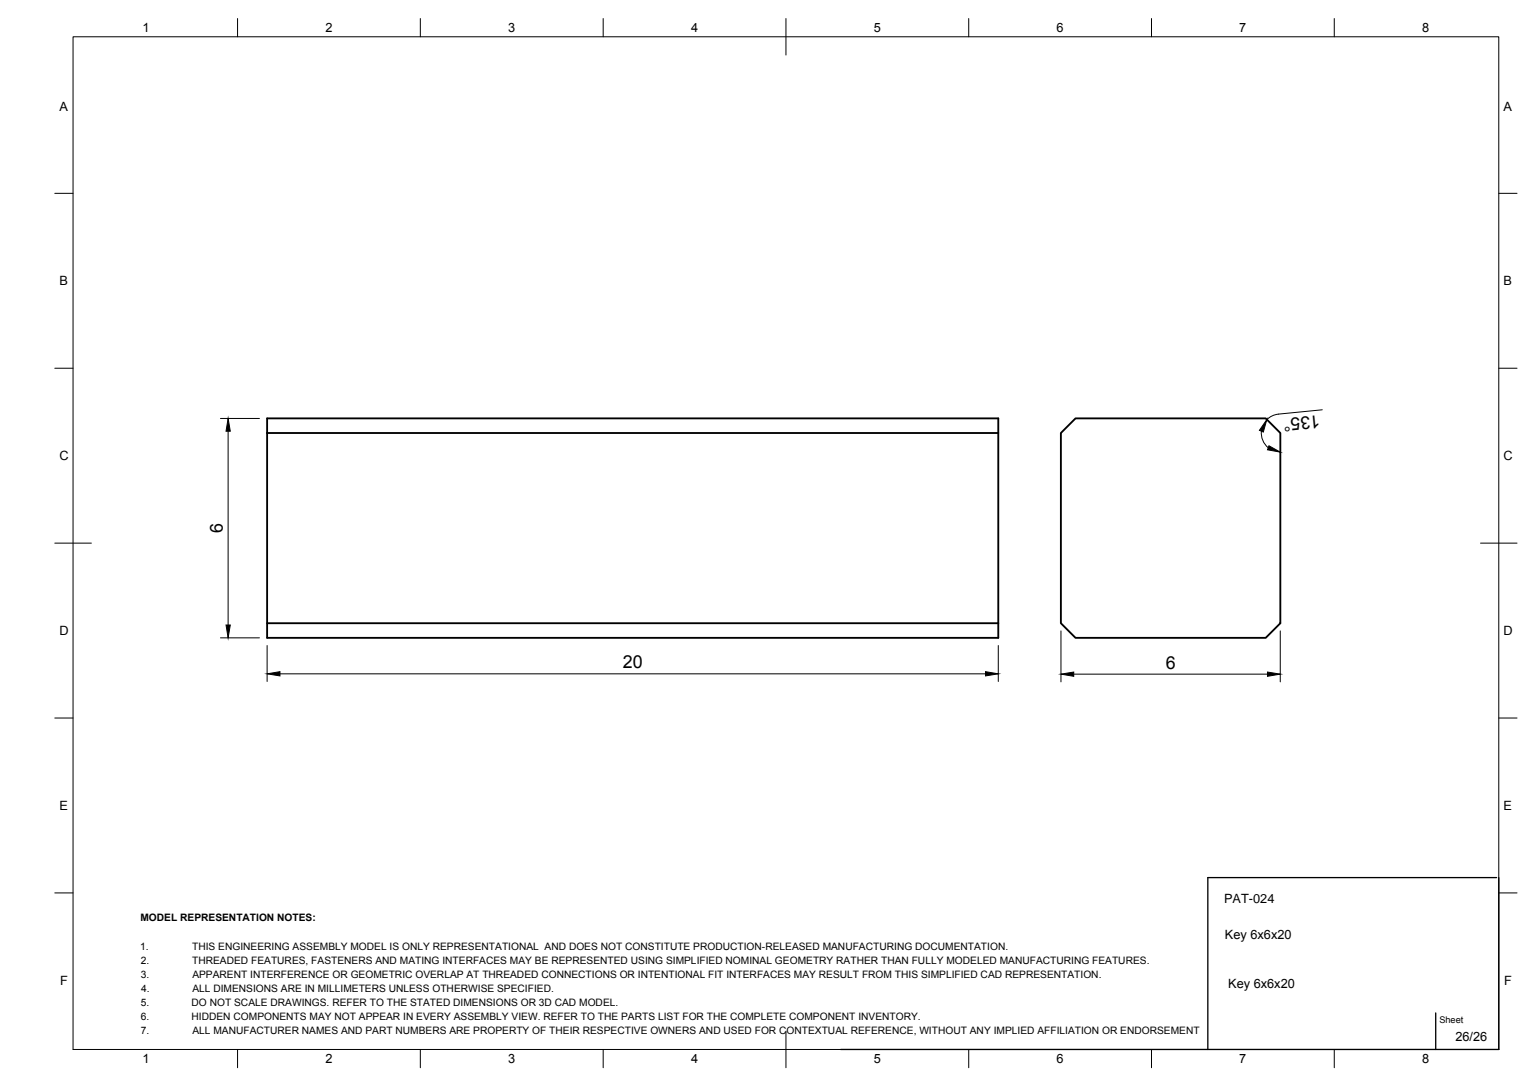
ISO-10303-21;
HEADER;
/* Generated by software containing ST-Developer
 * from STEP Tools, Inc. (www.steptools.com) 
 */

FILE_DESCRIPTION(
/* description */ ('Compact handwheel screw vise'),
/* implementation_level */ '2;1');

FILE_NAME(
/* name */ 'Key 6x6x20.step',
/* time_stamp */ '2026-10-29T16:08:22-07:00',
/* author */ (''),
/* organization */ (''),
/* preprocessor_version */ 'ST-DEVELOPER v20.2',
/* originating_system */ 'Autodesk Translation Framework v15.17.0.0',
/* authorisation */ '');

FILE_SCHEMA (('AUTOMOTIVE_DESIGN { 1 0 10303 214 3 1 1 }'));
ENDSEC;

DATA;
#10=MECHANICAL_DESIGN_GEOMETRIC_PRESENTATION_REPRESENTATION('',(#676),#25074);
#612=SHAPE_REPRESENTATION_RELATIONSHIP('SRR','None',#25223,#640);
#640=ADVANCED_BREP_SHAPE_REPRESENTATION('',(#709),#25070);
#676=STYLED_ITEM('',(#25439),#709);
#709=MANIFOLD_SOLID_BREP('Body1',#8087);
#980=PLANE('',#9109);
#981=PLANE('',#9110);
#982=PLANE('',#9111);
#983=PLANE('',#9112);
#984=PLANE('',#9113);
#985=PLANE('',#9114);
#986=PLANE('',#9115);
#987=PLANE('',#9116);
#988=PLANE('',#9117);
#989=PLANE('',#9118);
#1439=FACE_OUTER_BOUND('',#2015,.T.);
#1440=FACE_OUTER_BOUND('',#2016,.T.);
#1441=FACE_OUTER_BOUND('',#2017,.T.);
#1442=FACE_OUTER_BOUND('',#2018,.T.);
#1443=FACE_OUTER_BOUND('',#2019,.T.);
#1444=FACE_OUTER_BOUND('',#2020,.T.);
#1445=FACE_OUTER_BOUND('',#2021,.T.);
#1446=FACE_OUTER_BOUND('',#2022,.T.);
#1447=FACE_OUTER_BOUND('',#2023,.T.);
#1448=FACE_OUTER_BOUND('',#2024,.T.);
#2015=EDGE_LOOP('',(#7171,#7172,#7173,#7174,#7175,#7176,#7177,#7178));
#2016=EDGE_LOOP('',(#7179,#7180,#7181,#7182));
#2017=EDGE_LOOP('',(#7183,#7184,#7185,#7186));
#2018=EDGE_LOOP('',(#7187,#7188,#7189,#7190));
#2019=EDGE_LOOP('',(#7191,#7192,#7193,#7194));
#2020=EDGE_LOOP('',(#7195,#7196,#7197,#7198,#7199,#7200,#7201,#7202));
#2021=EDGE_LOOP('',(#7203,#7204,#7205,#7206));
#2022=EDGE_LOOP('',(#7207,#7208,#7209,#7210));
#2023=EDGE_LOOP('',(#7211,#7212,#7213,#7214));
#2024=EDGE_LOOP('',(#7215,#7216,#7217,#7218));
#2499=LINE('',#24788,#3007);
#2500=LINE('',#24790,#3008);
#2501=LINE('',#24792,#3009);
#2502=LINE('',#24794,#3010);
#2503=LINE('',#24796,#3011);
#2504=LINE('',#24798,#3012);
#2505=LINE('',#24800,#3013);
#2506=LINE('',#24801,#3014);
#2507=LINE('',#24804,#3015);
#2508=LINE('',#24806,#3016);
#2509=LINE('',#24807,#3017);
#2510=LINE('',#24810,#3018);
#2511=LINE('',#24811,#3019);
#2512=LINE('',#24814,#3020);
#2513=LINE('',#24815,#3021);
#2514=LINE('',#24818,#3022);
#2515=LINE('',#24819,#3023);
#2516=LINE('',#24823,#3024);
#2517=LINE('',#24824,#3025);
#2518=LINE('',#24826,#3026);
#2519=LINE('',#24827,#3027);
#2520=LINE('',#24829,#3028);
#2521=LINE('',#24831,#3029);
#2522=LINE('',#24833,#3030);
#3007=VECTOR('',#11059,1.);
#3008=VECTOR('',#11060,1.);
#3009=VECTOR('',#11061,1.);
#3010=VECTOR('',#11062,1.);
#3011=VECTOR('',#11063,1.);
#3012=VECTOR('',#11064,1.);
#3013=VECTOR('',#11065,1.);
#3014=VECTOR('',#11066,1.);
#3015=VECTOR('',#11069,1.);
#3016=VECTOR('',#11070,1.);
#3017=VECTOR('',#11071,1.);
#3018=VECTOR('',#11074,1.);
#3019=VECTOR('',#11075,1.);
#3020=VECTOR('',#11078,1.);
#3021=VECTOR('',#11079,1.);
#3022=VECTOR('',#11082,1.);
#3023=VECTOR('',#11083,1.);
#3024=VECTOR('',#11086,1.);
#3025=VECTOR('',#11087,1.);
#3026=VECTOR('',#11088,1.);
#3027=VECTOR('',#11089,1.);
#3028=VECTOR('',#11092,1.);
#3029=VECTOR('',#11095,1.);
#3030=VECTOR('',#11098,1.);
#4010=VERTEX_POINT('',#24786);
#4011=VERTEX_POINT('',#24787);
#4012=VERTEX_POINT('',#24789);
#4013=VERTEX_POINT('',#24791);
#4014=VERTEX_POINT('',#24793);
#4015=VERTEX_POINT('',#24795);
#4016=VERTEX_POINT('',#24797);
#4017=VERTEX_POINT('',#24799);
#4018=VERTEX_POINT('',#24803);
#4019=VERTEX_POINT('',#24805);
#4020=VERTEX_POINT('',#24809);
#4021=VERTEX_POINT('',#24813);
#4022=VERTEX_POINT('',#24817);
#4023=VERTEX_POINT('',#24821);
#4024=VERTEX_POINT('',#24822);
#4025=VERTEX_POINT('',#24825);
#5072=EDGE_CURVE('',#4010,#4011,#2499,.T.);
#5073=EDGE_CURVE('',#4012,#4010,#2500,.T.);
#5074=EDGE_CURVE('',#4013,#4012,#2501,.T.);
#5075=EDGE_CURVE('',#4014,#4013,#2502,.T.);
#5076=EDGE_CURVE('',#4015,#4014,#2503,.T.);
#5077=EDGE_CURVE('',#4016,#4015,#2504,.T.);
#5078=EDGE_CURVE('',#4017,#4016,#2505,.T.);
#5079=EDGE_CURVE('',#4011,#4017,#2506,.T.);
#5080=EDGE_CURVE('',#4014,#4018,#2507,.T.);
#5081=EDGE_CURVE('',#4018,#4019,#2508,.T.);
#5082=EDGE_CURVE('',#4019,#4015,#2509,.T.);
#5083=EDGE_CURVE('',#4020,#4013,#2510,.T.);
#5084=EDGE_CURVE('',#4020,#4018,#2511,.T.);
#5085=EDGE_CURVE('',#4012,#4021,#2512,.T.);
#5086=EDGE_CURVE('',#4021,#4020,#2513,.T.);
#5087=EDGE_CURVE('',#4022,#4010,#2514,.T.);
#5088=EDGE_CURVE('',#4022,#4021,#2515,.T.);
#5089=EDGE_CURVE('',#4023,#4024,#2516,.T.);
#5090=EDGE_CURVE('',#4019,#4023,#2517,.T.);
#5091=EDGE_CURVE('',#4025,#4022,#2518,.T.);
#5092=EDGE_CURVE('',#4024,#4025,#2519,.T.);
#5093=EDGE_CURVE('',#4016,#4023,#2520,.T.);
#5094=EDGE_CURVE('',#4011,#4025,#2521,.T.);
#5095=EDGE_CURVE('',#4024,#4017,#2522,.T.);
#7171=ORIENTED_EDGE('',*,*,#5072,.F.);
#7172=ORIENTED_EDGE('',*,*,#5073,.F.);
#7173=ORIENTED_EDGE('',*,*,#5074,.F.);
#7174=ORIENTED_EDGE('',*,*,#5075,.F.);
#7175=ORIENTED_EDGE('',*,*,#5076,.F.);
#7176=ORIENTED_EDGE('',*,*,#5077,.F.);
#7177=ORIENTED_EDGE('',*,*,#5078,.F.);
#7178=ORIENTED_EDGE('',*,*,#5079,.F.);
#7179=ORIENTED_EDGE('',*,*,#5076,.T.);
#7180=ORIENTED_EDGE('',*,*,#5080,.T.);
#7181=ORIENTED_EDGE('',*,*,#5081,.T.);
#7182=ORIENTED_EDGE('',*,*,#5082,.T.);
#7183=ORIENTED_EDGE('',*,*,#5075,.T.);
#7184=ORIENTED_EDGE('',*,*,#5083,.F.);
#7185=ORIENTED_EDGE('',*,*,#5084,.T.);
#7186=ORIENTED_EDGE('',*,*,#5080,.F.);
#7187=ORIENTED_EDGE('',*,*,#5074,.T.);
#7188=ORIENTED_EDGE('',*,*,#5085,.T.);
#7189=ORIENTED_EDGE('',*,*,#5086,.T.);
#7190=ORIENTED_EDGE('',*,*,#5083,.T.);
#7191=ORIENTED_EDGE('',*,*,#5073,.T.);
#7192=ORIENTED_EDGE('',*,*,#5087,.F.);
#7193=ORIENTED_EDGE('',*,*,#5088,.T.);
#7194=ORIENTED_EDGE('',*,*,#5085,.F.);
#7195=ORIENTED_EDGE('',*,*,#5089,.F.);
#7196=ORIENTED_EDGE('',*,*,#5090,.F.);
#7197=ORIENTED_EDGE('',*,*,#5081,.F.);
#7198=ORIENTED_EDGE('',*,*,#5084,.F.);
#7199=ORIENTED_EDGE('',*,*,#5086,.F.);
#7200=ORIENTED_EDGE('',*,*,#5088,.F.);
#7201=ORIENTED_EDGE('',*,*,#5091,.F.);
#7202=ORIENTED_EDGE('',*,*,#5092,.F.);
#7203=ORIENTED_EDGE('',*,*,#5077,.T.);
#7204=ORIENTED_EDGE('',*,*,#5082,.F.);
#7205=ORIENTED_EDGE('',*,*,#5090,.T.);
#7206=ORIENTED_EDGE('',*,*,#5093,.F.);
#7207=ORIENTED_EDGE('',*,*,#5072,.T.);
#7208=ORIENTED_EDGE('',*,*,#5094,.T.);
#7209=ORIENTED_EDGE('',*,*,#5091,.T.);
#7210=ORIENTED_EDGE('',*,*,#5087,.T.);
#7211=ORIENTED_EDGE('',*,*,#5078,.T.);
#7212=ORIENTED_EDGE('',*,*,#5093,.T.);
#7213=ORIENTED_EDGE('',*,*,#5089,.T.);
#7214=ORIENTED_EDGE('',*,*,#5095,.T.);
#7215=ORIENTED_EDGE('',*,*,#5079,.T.);
#7216=ORIENTED_EDGE('',*,*,#5095,.F.);
#7217=ORIENTED_EDGE('',*,*,#5092,.T.);
#7218=ORIENTED_EDGE('',*,*,#5094,.F.);
#8009=ADVANCED_FACE('',(#1439),#980,.F.);
#8010=ADVANCED_FACE('',(#1440),#981,.T.);
#8011=ADVANCED_FACE('',(#1441),#982,.T.);
#8012=ADVANCED_FACE('',(#1442),#983,.T.);
#8013=ADVANCED_FACE('',(#1443),#984,.T.);
#8014=ADVANCED_FACE('',(#1444),#985,.T.);
#8015=ADVANCED_FACE('',(#1445),#986,.F.);
#8016=ADVANCED_FACE('',(#1446),#987,.T.);
#8017=ADVANCED_FACE('',(#1447),#988,.T.);
#8018=ADVANCED_FACE('',(#1448),#989,.T.);
#8087=CLOSED_SHELL('',(#8009,#8010,#8011,#8012,#8013,#8014,#8015,#8016,
#8017,#8018));
#9108=AXIS2_PLACEMENT_3D('',#24784,#11055,#11056);
#9109=AXIS2_PLACEMENT_3D('',#24785,#11057,#11058);
#9110=AXIS2_PLACEMENT_3D('',#24802,#11067,#11068);
#9111=AXIS2_PLACEMENT_3D('',#24808,#11072,#11073);
#9112=AXIS2_PLACEMENT_3D('',#24812,#11076,#11077);
#9113=AXIS2_PLACEMENT_3D('',#24816,#11080,#11081);
#9114=AXIS2_PLACEMENT_3D('',#24820,#11084,#11085);
#9115=AXIS2_PLACEMENT_3D('',#24828,#11090,#11091);
#9116=AXIS2_PLACEMENT_3D('',#24830,#11093,#11094);
#9117=AXIS2_PLACEMENT_3D('',#24832,#11096,#11097);
#9118=AXIS2_PLACEMENT_3D('',#24834,#11099,#11100);
#11055=DIRECTION('axis',(0.,0.,1.));
#11056=DIRECTION('refdir',(1.,0.,0.));
#11057=DIRECTION('center_axis',(1.,0.,0.));
#11058=DIRECTION('ref_axis',(0.,0.,-1.));
#11059=DIRECTION('',(0.,-0.707106781186547,-0.707106781186548));
#11060=DIRECTION('',(0.,-1.,0.));
#11061=DIRECTION('',(0.,-0.707106781186547,0.707106781186548));
#11062=DIRECTION('',(0.,0.,1.));
#11063=DIRECTION('',(0.,0.707106781186547,0.707106781186548));
#11064=DIRECTION('',(0.,1.,0.));
#11065=DIRECTION('',(0.,0.707106781186547,-0.707106781186548));
#11066=DIRECTION('',(0.,0.,-1.));
#11067=DIRECTION('center_axis',(0.,0.707106781186548,-0.707106781186547));
#11068=DIRECTION('ref_axis',(-1.,0.,0.));
#11069=DIRECTION('',(1.,0.,0.));
#11070=DIRECTION('',(0.,-0.707106781186547,-0.707106781186548));
#11071=DIRECTION('',(-1.,0.,0.));
#11072=DIRECTION('center_axis',(0.,1.,0.));
#11073=DIRECTION('ref_axis',(-1.,0.,0.));
#11074=DIRECTION('',(-1.,0.,0.));
#11075=DIRECTION('',(0.,0.,-1.));
#11076=DIRECTION('center_axis',(0.,0.707106781186548,0.707106781186547));
#11077=DIRECTION('ref_axis',(1.,0.,0.));
#11078=DIRECTION('',(1.,0.,0.));
#11079=DIRECTION('',(0.,0.707106781186547,-0.707106781186548));
#11080=DIRECTION('center_axis',(0.,0.,1.));
#11081=DIRECTION('ref_axis',(1.,0.,0.));
#11082=DIRECTION('',(-1.,0.,0.));
#11083=DIRECTION('',(0.,1.,0.));
#11084=DIRECTION('center_axis',(1.,0.,0.));
#11085=DIRECTION('ref_axis',(0.,0.,-1.));
#11086=DIRECTION('',(0.,-0.707106781186547,0.707106781186548));
#11087=DIRECTION('',(0.,-1.,0.));
#11088=DIRECTION('',(0.,0.707106781186547,0.707106781186548));
#11089=DIRECTION('',(0.,0.,1.));
#11090=DIRECTION('center_axis',(0.,0.,1.));
#11091=DIRECTION('ref_axis',(1.,0.,0.));
#11092=DIRECTION('',(1.,0.,0.));
#11093=DIRECTION('center_axis',(0.,-0.707106781186548,0.707106781186547));
#11094=DIRECTION('ref_axis',(1.,0.,0.));
#11095=DIRECTION('',(1.,0.,0.));
#11096=DIRECTION('center_axis',(0.,-0.707106781186548,-0.707106781186547));
#11097=DIRECTION('ref_axis',(-1.,0.,0.));
#11098=DIRECTION('',(-1.,0.,0.));
#11099=DIRECTION('center_axis',(0.,-1.,0.));
#11100=DIRECTION('ref_axis',(1.,0.,0.));
#24784=CARTESIAN_POINT('',(0.,0.,0.));
#24785=CARTESIAN_POINT('Origin',(-1.,0.,0.35));
#24786=CARTESIAN_POINT('',(-1.,-0.26,0.6));
#24787=CARTESIAN_POINT('',(-1.,-0.3,0.56));
#24788=CARTESIAN_POINT('',(-1.,-0.2675,0.5925));
#24789=CARTESIAN_POINT('',(-1.,0.26,0.6));
#24790=CARTESIAN_POINT('',(-1.,0.,0.6));
#24791=CARTESIAN_POINT('',(-1.,0.3,0.56));
#24792=CARTESIAN_POINT('',(-1.,0.2675,0.5925));
#24793=CARTESIAN_POINT('',(-1.,0.3,0.04));
#24794=CARTESIAN_POINT('',(-1.,0.3,0.175));
#24795=CARTESIAN_POINT('',(-1.,0.26,0.));
#24796=CARTESIAN_POINT('',(-1.,0.2925,0.0325));
#24797=CARTESIAN_POINT('',(-1.,-0.26,0.));
#24798=CARTESIAN_POINT('',(-1.,0.,0.));
#24799=CARTESIAN_POINT('',(-1.,-0.3,0.04));
#24800=CARTESIAN_POINT('',(-1.,-0.2925,0.0325));
#24801=CARTESIAN_POINT('',(-1.,-0.3,0.175));
#24802=CARTESIAN_POINT('Origin',(0.75,0.28,0.02));
#24803=CARTESIAN_POINT('',(1.,0.3,0.04));
#24804=CARTESIAN_POINT('',(0.75,0.3,0.04));
#24805=CARTESIAN_POINT('',(1.,0.26,0.));
#24806=CARTESIAN_POINT('',(1.,0.2925,0.0325));
#24807=CARTESIAN_POINT('',(0.75,0.26,0.));
#24808=CARTESIAN_POINT('Origin',(1.5,0.3,0.));
#24809=CARTESIAN_POINT('',(1.,0.3,0.56));
#24810=CARTESIAN_POINT('',(0.75,0.3,0.56));
#24811=CARTESIAN_POINT('',(1.,0.3,0.175));
#24812=CARTESIAN_POINT('Origin',(0.75,0.28,0.58));
#24813=CARTESIAN_POINT('',(1.,0.26,0.6));
#24814=CARTESIAN_POINT('',(0.75,0.26,0.6));
#24815=CARTESIAN_POINT('',(1.,0.2675,0.5925));
#24816=CARTESIAN_POINT('Origin',(0.,0.,0.6));
#24817=CARTESIAN_POINT('',(1.,-0.26,0.6));
#24818=CARTESIAN_POINT('',(-0.75,-0.26,0.6));
#24819=CARTESIAN_POINT('',(1.,0.,0.6));
#24820=CARTESIAN_POINT('Origin',(1.,0.,0.35));
#24821=CARTESIAN_POINT('',(1.,-0.26,0.));
#24822=CARTESIAN_POINT('',(1.,-0.3,0.04));
#24823=CARTESIAN_POINT('',(1.,-0.2925,0.0325));
#24824=CARTESIAN_POINT('',(1.,0.,0.));
#24825=CARTESIAN_POINT('',(1.,-0.3,0.56));
#24826=CARTESIAN_POINT('',(1.,-0.2675,0.5925));
#24827=CARTESIAN_POINT('',(1.,-0.3,0.175));
#24828=CARTESIAN_POINT('Origin',(0.,0.,0.));
#24829=CARTESIAN_POINT('',(-0.75,-0.26,0.));
#24830=CARTESIAN_POINT('Origin',(-0.75,-0.28,0.58));
#24831=CARTESIAN_POINT('',(-0.75,-0.3,0.56));
#24832=CARTESIAN_POINT('Origin',(-0.75,-0.28,0.02));
#24833=CARTESIAN_POINT('',(-0.75,-0.3,0.04));
#24834=CARTESIAN_POINT('Origin',(-1.5,-0.3,0.));
#25036=UNCERTAINTY_MEASURE_WITH_UNIT(LENGTH_MEASURE(0.001),#25075,
'DISTANCE_ACCURACY_VALUE',
'Maximum model space distance between geometric entities at asserted c
onnectivities');
#25040=UNCERTAINTY_MEASURE_WITH_UNIT(LENGTH_MEASURE(0.001),#25075,
'DISTANCE_ACCURACY_VALUE',
'Maximum model space distance between geometric entities at asserted c
onnectivities');
#25070=(
GEOMETRIC_REPRESENTATION_CONTEXT(3)
GLOBAL_UNCERTAINTY_ASSIGNED_CONTEXT((#25036))
GLOBAL_UNIT_ASSIGNED_CONTEXT((#25075,#25077,#25078))
REPRESENTATION_CONTEXT('','3D')
);
#25074=(
GEOMETRIC_REPRESENTATION_CONTEXT(3)
GLOBAL_UNCERTAINTY_ASSIGNED_CONTEXT((#25040))
GLOBAL_UNIT_ASSIGNED_CONTEXT((#25075,#25077,#25078))
REPRESENTATION_CONTEXT('','3D')
);
#25075=(
LENGTH_UNIT()
NAMED_UNIT(*)
SI_UNIT(.CENTI.,.METRE.)
);
#25077=(
NAMED_UNIT(*)
PLANE_ANGLE_UNIT()
SI_UNIT($,.RADIAN.)
);
#25078=(
NAMED_UNIT(*)
SI_UNIT($,.STERADIAN.)
SOLID_ANGLE_UNIT()
);
#25108=SHAPE_DEFINITION_REPRESENTATION(#25157,#25223);
#25157=PRODUCT_DEFINITION_SHAPE('',$,#25257);
#25223=SHAPE_REPRESENTATION('',(#9108),#25070);
#25227=PRODUCT_DEFINITION_CONTEXT('part definition',#25328,'design');
#25257=PRODUCT_DEFINITION('Key 6x6x20','Key 6x6x20',#25290,#25227);
#25290=PRODUCT_DEFINITION_FORMATION('',$,#25359);
#25328=APPLICATION_CONTEXT(
'Core Data for Automotive Mechanical Design Process');
#25329=PRODUCT_CONTEXT('part definition',#25328,'mechanical');
#25359=PRODUCT('Key 6x6x20','Key 6x6x20','Key 6x6x20',(#25329));
#25433=COLOUR_RGB('Grey',0.48,0.52,0.57);
#25434=FILL_AREA_STYLE_COLOUR('',#25433);
#25435=FILL_AREA_STYLE('',(#25434));
#25436=SURFACE_STYLE_FILL_AREA(#25435);
#25437=SURFACE_SIDE_STYLE('',(#25436));
#25438=SURFACE_STYLE_USAGE(.BOTH.,#25437);
#25439=PRESENTATION_STYLE_ASSIGNMENT((#25438));
ENDSEC;
END-ISO-10303-21;
